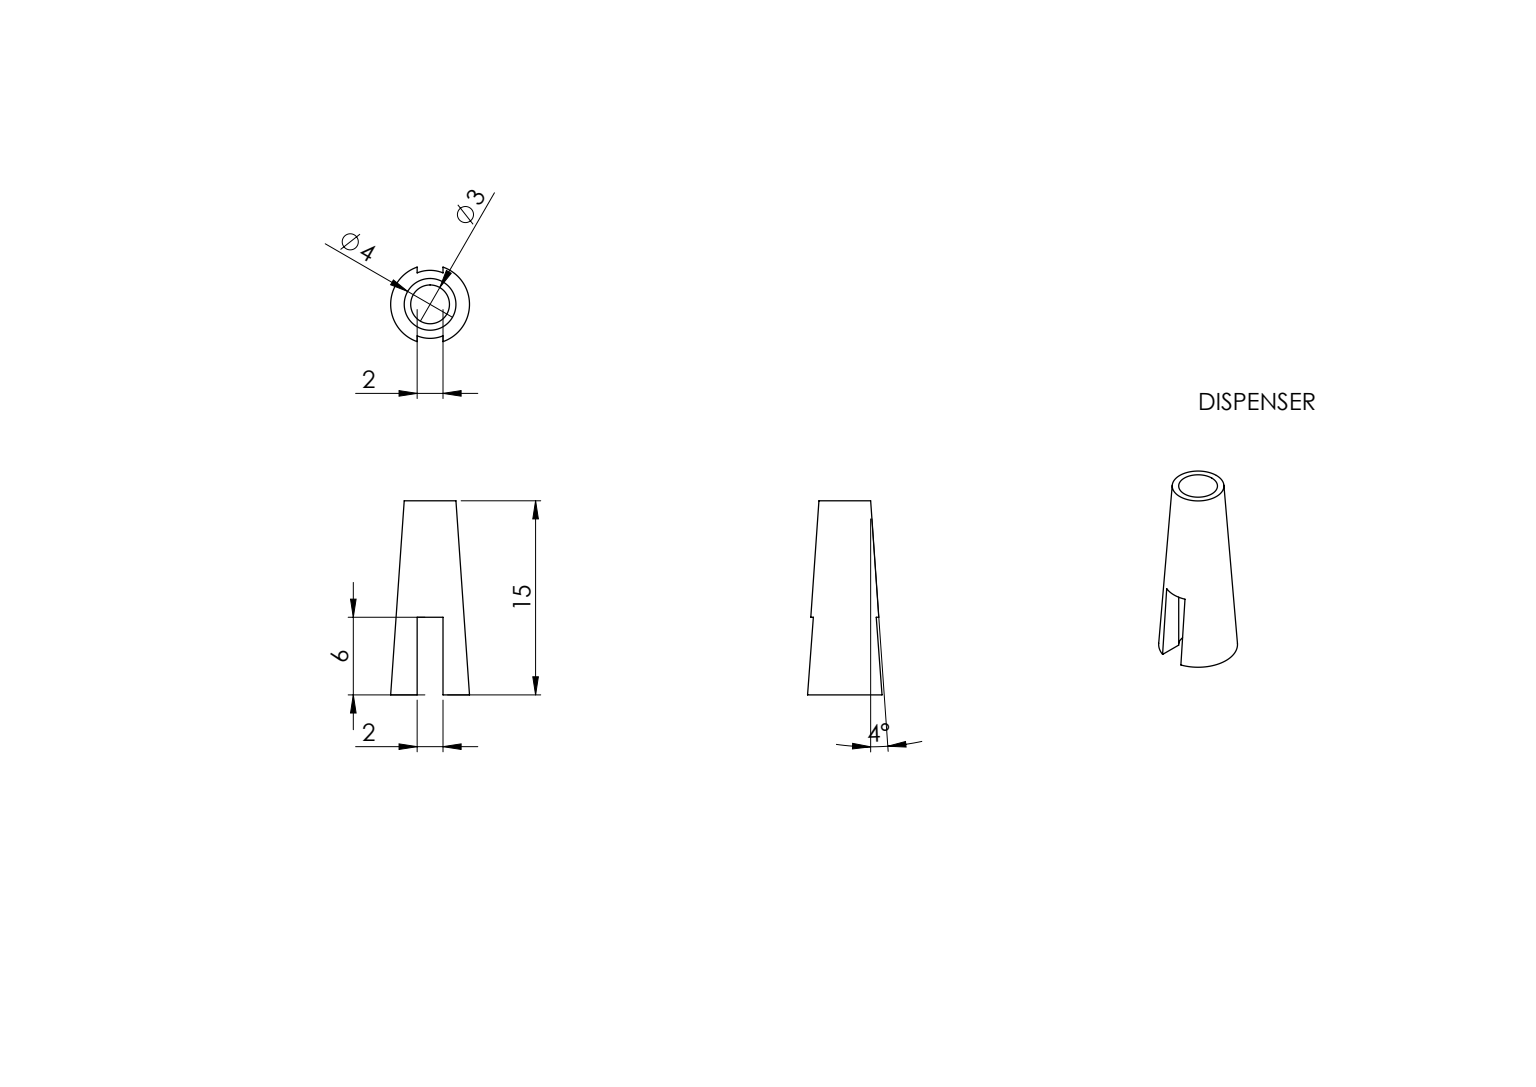
ISO-10303-21;
HEADER;
FILE_DESCRIPTION (('STEP AP214'),
    '1' );
FILE_NAME ('dispenser.step',
    '2026-10-27T10:49:47',
    ( '' ),
    ( '' ),
    'SwSTEP 2.0',
    'SolidWorks 2026',
    '' );
FILE_SCHEMA (( 'AUTOMOTIVE_DESIGN' ));
ENDSEC;

DATA;
#7=CARTESIAN_POINT ( 'NONE',  ( 1.000000000000000000, -30.99987166532831395, 2.582963027349738816 ) ) ;
#10=VECTOR ( 'NONE', #8817, 1000.000000000000000 ) ;
#30=CARTESIAN_POINT ( 'NONE',  ( -1.000000000000000000, -29.00000000000000355, -1.118033988749894680 ) ) ;
#57=DIRECTION ( 'NONE',  ( 0.000000000000000000, 0.000000000000000000, -1.000000000000000000 ) ) ;
#70=CARTESIAN_POINT ( 'NONE',  ( 1.000000000000000000, -29.00000000000000355, -2.431755684948965435 ) ) ;
#75=LINE ( 'NONE', #5700, #8771 ) ;
#80=DIRECTION ( 'NONE',  ( 0.000000000000000000, 0.000000000000000000, -1.000000000000000000 ) ) ;
#99=PRODUCT_DEFINITION_SHAPE ( 'NONE', 'NONE',  #1543 ) ;
#107=CARTESIAN_POINT ( 'NONE',  ( 0.000000000000000000, -29.00000000000000355, -1.499999999999999778 ) ) ;
#115=CARTESIAN_POINT ( 'NONE',  ( 1.836970198721029688E-16, -29.00000000000000355, 1.499999999999999778 ) ) ;
#120=UNCERTAINTY_MEASURE_WITH_UNIT (LENGTH_MEASURE( 1.000000000000000082E-05 ), #327, 'distance_accuracy_value', 'NONE');
#123=CIRCLE ( 'NONE', #1315, 2.629341307491595447 ) ;
#134=FACE_OUTER_BOUND ( 'NONE', #6393, .T. ) ;
#153=DIRECTION ( 'NONE',  ( 1.000000000000000000, 0.000000000000000000, 0.000000000000000000 ) ) ;
#178=DIRECTION ( 'NONE',  ( 0.000000000000000000, -1.000000000000000000, 0.000000000000000000 ) ) ;
#228=FACE_OUTER_BOUND ( 'NONE', #8574, .T. ) ;
#277=ORIENTED_EDGE ( 'NONE', *, *, #3202, .T. ) ;
#282=AXIS2_PLACEMENT_3D ( 'NONE', #7052, #2786, #2167 ) ;
#327=( LENGTH_UNIT ( ) NAMED_UNIT ( * ) SI_UNIT ( .MILLI., .METRE. ) );
#344=AXIS2_PLACEMENT_3D ( 'NONE', #6374, #8568, #2197 ) ;
#388=EDGE_LOOP ( 'NONE', ( #5734, #5832, #6280, #502 ) ) ;
#501=( GEOMETRIC_REPRESENTATION_CONTEXT ( 3 ) GLOBAL_UNCERTAINTY_ASSIGNED_CONTEXT ( ( #1749 ) ) GLOBAL_UNIT_ASSIGNED_CONTEXT ( ( #4938, #8573, #8161 ) ) REPRESENTATION_CONTEXT ( 'NONE', 'WORKASPACE' ) );
#502=ORIENTED_EDGE ( 'NONE', *, *, #1398, .F. ) ;
#521=DIRECTION ( 'NONE',  ( 0.000000000000000000, 0.000000000000000000, -1.000000000000000000 ) ) ;
#574=VECTOR ( 'NONE', #6967, 1000.000000000000000 ) ;
#647=AXIS2_PLACEMENT_3D ( 'NONE', #4691, #1868, #7487 ) ;
#652=EDGE_CURVE ( 'NONE', #8139, #3081, #2009, .T. ) ;
#656=ORIENTED_EDGE ( 'NONE', *, *, #6309, .F. ) ;
#677=ORIENTED_EDGE ( 'NONE', *, *, #5454, .F. ) ;
#678=CARTESIAN_POINT ( 'NONE',  ( -1.000000000000000000, -20.00000000000000000, 1.118033988749894680 ) ) ;
#699=( GEOMETRIC_REPRESENTATION_CONTEXT ( 3 ) GLOBAL_UNCERTAINTY_ASSIGNED_CONTEXT ( ( #120 ) ) GLOBAL_UNIT_ASSIGNED_CONTEXT ( ( #327, #6002, #8152 ) ) REPRESENTATION_CONTEXT ( 'NONE', 'WORKASPACE' ) );
#702=DIRECTION ( 'NONE',  ( 0.000000000000000000, 0.000000000000000000, -1.000000000000000000 ) ) ;
#718=LINE ( 'NONE', #5695, #7261 ) ;
#720=ORIENTED_EDGE ( 'NONE', *, *, #7534, .F. ) ;
#721=DIRECTION ( 'NONE',  ( -0.000000000000000000, -0.000000000000000000, 1.000000000000000000 ) ) ;
#723=DIRECTION ( 'NONE',  ( 1.000000000000000000, 0.000000000000000000, 0.000000000000000000 ) ) ;
#742=CONICAL_SURFACE ( 'NONE', #6530, 2.000000000000000000, 0.06981317007977333455 ) ;
#762=ORIENTED_EDGE ( 'NONE', *, *, #2487, .F. ) ;
#783=EDGE_CURVE ( 'NONE', #3636, #7860, #7922, .T. ) ;
#852=ORIENTED_EDGE ( 'NONE', *, *, #1586, .F. ) ;
#873=CARTESIAN_POINT ( 'NONE',  ( 0.000000000000000000, -29.00000000000000355, 0.000000000000000000 ) ) ;
#883=ORIENTED_EDGE ( 'NONE', *, *, #8729, .F. ) ;
#888=AXIS2_PLACEMENT_3D ( 'NONE', #4026, #9081, #6861 ) ;
#894=CARTESIAN_POINT ( 'NONE',  ( -1.000000000000000000, -30.99987166532831395, 2.582963027349738816 ) ) ;
#950=DIRECTION ( 'NONE',  ( 0.000000000000000000, -1.000000000000000000, 0.000000000000000000 ) ) ;
#997=CARTESIAN_POINT ( 'NONE',  ( -1.000000000000000000, -29.00000000000000355, -3.048902179152658931 ) ) ;
#1022=ORIENTED_EDGE ( 'NONE', *, *, #4471, .T. ) ;
#1029=EDGE_LOOP ( 'NONE', ( #277, #4373, #5520, #6752, #7836, #4879, #5582, #4542 ) ) ;
#1102=DIRECTION ( 'NONE',  ( 0.000000000000000000, -1.000000000000000000, 0.000000000000000000 ) ) ;
#1137=CARTESIAN_POINT ( 'NONE',  ( 0.000000000000000000, -35.00000000000000000, 0.000000000000000000 ) ) ;
#1194=AXIS2_PLACEMENT_3D ( 'NONE', #7137, #7046, #3559 ) ;
#1208=DIRECTION ( 'NONE',  ( 0.000000000000000000, -0.000000000000000000, -1.000000000000000000 ) ) ;
#1241=DIRECTION ( 'NONE',  ( 0.000000000000000000, 0.000000000000000000, -1.000000000000000000 ) ) ;
#1282=EDGE_LOOP ( 'NONE', ( #7453, #8242, #8885, #677 ) ) ;
#1286=VERTEX_POINT ( 'NONE', #30 ) ;
#1307=EDGE_CURVE ( 'NONE', #6715, #7860, #2924, .T. ) ;
#1315=AXIS2_PLACEMENT_3D ( 'NONE', #2177, #2930, #80 ) ;
#1338=AXIS2_PLACEMENT_3D ( 'NONE', #873, #178, #3771 ) ;
#1360=ADVANCED_FACE ( 'NONE', ( #4178, #2747 ), #7806, .F. ) ;
#1387=DIRECTION ( 'NONE',  ( 0.000000000000000000, -0.000000000000000000, -1.000000000000000000 ) ) ;
#1392=CARTESIAN_POINT ( 'NONE',  ( 1.000000000000000000, -29.00000000000000355, 1.118033988749894680 ) ) ;
#1398=EDGE_CURVE ( 'NONE', #6849, #8000, #8214, .T. ) ;
#1409=PLANE ( 'NONE',  #344 ) ;
#1420=DIRECTION ( 'NONE',  ( -0.000000000000000000, -0.000000000000000000, 1.000000000000000000 ) ) ;
#1442=EDGE_CURVE ( 'NONE', #1286, #7860, #7941, .T. ) ;
#1448=CARTESIAN_POINT ( 'NONE',  ( -1.000000000000000000, -35.00000000000000000, -2.880243826144208708 ) ) ;
#1466=CARTESIAN_POINT ( 'NONE',  ( 1.000000000000000000, -35.00000000000000000, -2.880243826144208708 ) ) ;
#1497=DIRECTION ( 'NONE',  ( 0.000000000000000000, 0.000000000000000000, -1.000000000000000000 ) ) ;
#1498=CARTESIAN_POINT ( 'NONE',  ( -1.000000000000000000, -35.00000000000000000, 2.880243826144208708 ) ) ;
#1514=CARTESIAN_POINT ( 'NONE',  ( -1.000000000000000000, -35.00000000000000000, -3.048902179152658931 ) ) ;
#1543=PRODUCT_DEFINITION ( 'UNKNOWN', '', #8579, #8974 ) ;
#1586=EDGE_CURVE ( 'NONE', #7256, #3429, #6249, .T. ) ;
#1590=CARTESIAN_POINT ( 'NONE',  ( 1.000000000000000000, -35.00000000000000000, -1.118033988749894680 ) ) ;
#1591=DIRECTION ( 'NONE',  ( 8.542704229054961664E-18, -0.9975640502598241977, 0.06975647374412545509 ) ) ;
#1637=AXIS2_PLACEMENT_3D ( 'NONE', #1137, #4623, #5581 ) ;
#1638=CARTESIAN_POINT ( 'NONE',  ( 0.000000000000000000, -29.00000000000000355, 0.000000000000000000 ) ) ;
#1644=FACE_OUTER_BOUND ( 'NONE', #1282, .T. ) ;
#1695=DIRECTION ( 'NONE',  ( 1.000000000000000000, 0.000000000000000000, 0.000000000000000000 ) ) ;
#1714=DIRECTION ( 'NONE',  ( 0.000000000000000000, -1.000000000000000000, 0.000000000000000000 ) ) ;
#1749=UNCERTAINTY_MEASURE_WITH_UNIT (LENGTH_MEASURE( 1.000000000000000082E-05 ), #4938, 'distance_accuracy_value', 'NONE');
#1827=SHAPE_REPRESENTATION_RELATIONSHIP ( 'NONE' , 'NONE' ,  #1843, #2088 ) ;
#1834=CYLINDRICAL_SURFACE ( 'NONE', #6978, 1.499999999999999778 ) ;
#1841=CARTESIAN_POINT ( 'NONE',  ( 0.000000000000000000, -20.00000000000000000, 0.000000000000000000 ) ) ;
#1843=SHAPE_REPRESENTATION ( 'dispenser', ( #888 ), #699 ) ;
#1868=DIRECTION ( 'NONE',  ( 0.000000000000000000, -1.000000000000000000, 0.000000000000000000 ) ) ;
#1888=EDGE_CURVE ( 'NONE', #7866, #8580, #8382, .T. ) ;
#1894=CARTESIAN_POINT ( 'NONE',  ( 0.000000000000000000, -20.00000000000000000, 0.000000000000000000 ) ) ;
#1905=MECHANICAL_DESIGN_GEOMETRIC_PRESENTATION_REPRESENTATION('',(#9023),#3833);
#1915=EDGE_CURVE ( 'NONE', #4653, #8235, #4037, .T. ) ;
#1921=DIRECTION ( 'NONE',  ( -0.000000000000000000, -1.000000000000000000, -0.000000000000000000 ) ) ;
#1943=VERTEX_POINT ( 'NONE', #6193 ) ;
#1944=CARTESIAN_POINT ( 'NONE',  ( 0.000000000000000000, -35.00000000000000000, 0.000000000000000000 ) ) ;
#1967=VERTEX_POINT ( 'NONE', #5393 ) ;
#1988=B_SPLINE_CURVE_WITH_KNOTS ( 'NONE', 3,
 ( #6414, #7, #8480, #2810 ),
 .UNSPECIFIED., .F., .F.,
 ( 4, 4 ),
 ( 0.008580651465885628590, 0.01459740681124464291 ),
 .UNSPECIFIED. ) ;
#2009=LINE ( 'NONE', #3362, #3473 ) ;
#2012=SURFACE_STYLE_USAGE ( .BOTH. , #6196 ) ;
#2024=FACE_OUTER_BOUND ( 'NONE', #4217, .T. ) ;
#2088=ADVANCED_BREP_SHAPE_REPRESENTATION ( '', ( #5133, #888 ), #699 ) ;
#2117=VERTEX_POINT ( 'NONE', #2933 ) ;
#2142=VERTEX_POINT ( 'NONE', #1392 ) ;
#2167=DIRECTION ( 'NONE',  ( 0.000000000000000000, 0.000000000000000000, -1.000000000000000000 ) ) ;
#2177=CARTESIAN_POINT ( 'NONE',  ( 0.000000000000000000, -29.00000000000000355, 0.000000000000000000 ) ) ;
#2197=DIRECTION ( 'NONE',  ( 0.000000000000000000, -0.000000000000000000, -1.000000000000000000 ) ) ;
#2198=CARTESIAN_POINT ( 'NONE',  ( 0.000000000000000000, -29.00000000000000355, 0.000000000000000000 ) ) ;
#2211=CARTESIAN_POINT ( 'NONE',  ( 0.000000000000000000, -20.00000000000000000, -1.499999999999999778 ) ) ;
#2221=DIRECTION ( 'NONE',  ( -0.000000000000000000, -0.000000000000000000, 1.000000000000000000 ) ) ;
#2228=CIRCLE ( 'NONE', #3431, 2.629341307491595447 ) ;
#2232=ORIENTED_EDGE ( 'NONE', *, *, #9006, .T. ) ;
#2300=PLANE ( 'NONE',  #4310 ) ;
#2321=CARTESIAN_POINT ( 'NONE',  ( -1.000000000000000000, -35.00000000000000000, 1.118033988749894458 ) ) ;
#2355=CARTESIAN_POINT ( 'NONE',  ( 1.836970198721029688E-16, -20.00000000000000000, 1.499999999999999778 ) ) ;
#2369=EDGE_CURVE ( 'NONE', #3636, #4653, #5653, .T. ) ;
#2370=DIRECTION ( 'NONE',  ( 1.000000000000000000, 0.000000000000000000, 0.000000000000000000 ) ) ;
#2384=CIRCLE ( 'NONE', #1637, 1.499999999999999778 ) ;
#2391=ORIENTED_EDGE ( 'NONE', *, *, #1915, .T. ) ;
#2393=AXIS2_PLACEMENT_3D ( 'NONE', #4264, #5741, #6395 ) ;
#2440=PLANE ( 'NONE',  #3474 ) ;
#2442=ORIENTED_EDGE ( 'NONE', *, *, #1307, .T. ) ;
#2487=EDGE_CURVE ( 'NONE', #6849, #8580, #7097, .T. ) ;
#2550=PLANE ( 'NONE',  #8924 ) ;
#2563=B_SPLINE_CURVE_WITH_KNOTS ( 'NONE', 3,
 ( #6467, #894, #4530, #1498 ),
 .UNSPECIFIED., .F., .F.,
 ( 4, 4 ),
 ( 0.008580651465885628590, 0.01459740681124464291 ),
 .UNSPECIFIED. ) ;
#2579=CONICAL_SURFACE ( 'NONE', #6132, 2.000000000000000000, 0.06981317007977333455 ) ;
#2605=EDGE_CURVE ( 'NONE', #3879, #8235, #2967, .T. ) ;
#2606=ORIENTED_EDGE ( 'NONE', *, *, #5013, .T. ) ;
#2614=PLANE ( 'NONE',  #4076 ) ;
#2629=ORIENTED_EDGE ( 'NONE', *, *, #6612, .T. ) ;
#2645=CARTESIAN_POINT ( 'NONE',  ( 0.000000000000000000, -29.00000000000000355, -2.629341307491595447 ) ) ;
#2670=FILL_AREA_STYLE ('',( #4706 ) ) ;
#2679=CARTESIAN_POINT ( 'NONE',  ( 0.000000000000000000, -20.00000000000000000, 0.000000000000000000 ) ) ;
#2681=FACE_OUTER_BOUND ( 'NONE', #1029, .T. ) ;
#2686=CLOSED_SHELL ( 'NONE', ( #8780, #4900, #2740, #3301, #7354, #1360, #6740, #5728, #3114, #3810, #5162, #9032, #5050 ) ) ;
#2713=VERTEX_POINT ( 'NONE', #2645 ) ;
#2740=ADVANCED_FACE ( 'NONE', ( #8267 ), #2550, .T. ) ;
#2747=FACE_OUTER_BOUND ( 'NONE', #6001, .T. ) ;
#2778=EDGE_CURVE ( 'NONE', #6849, #1943, #8193, .T. ) ;
#2786=DIRECTION ( 'NONE',  ( 0.000000000000000000, -1.000000000000000000, 0.000000000000000000 ) ) ;
#2810=CARTESIAN_POINT ( 'NONE',  ( 1.000000000000000000, -35.00000000000000000, 2.880243826144208708 ) ) ;
#2891=CIRCLE ( 'NONE', #647, 1.499999999999999778 ) ;
#2893=DIRECTION ( 'NONE',  ( -8.881784197001252323E-16, 0.000000000000000000, -1.000000000000000000 ) ) ;
#2896=EDGE_LOOP ( 'NONE', ( #2606, #5966, #5717, #4939 ) ) ;
#2904=APPLICATION_CONTEXT ( 'automotive_design' ) ;
#2924=LINE ( 'NONE', #1514, #574 ) ;
#2925=CARTESIAN_POINT ( 'NONE',  ( 1.000000000000000000, -35.00000000000000000, -3.048902179152658931 ) ) ;
#2930=DIRECTION ( 'NONE',  ( 0.000000000000000000, -1.000000000000000000, 0.000000000000000000 ) ) ;
#2933=CARTESIAN_POINT ( 'NONE',  ( 1.000000000000000000, -35.00000000000000000, 1.118033988749894680 ) ) ;
#2967=LINE ( 'NONE', #2355, #4889 ) ;
#2980=AXIS2_PLACEMENT_3D ( 'NONE', #4346, #5174, #4534 ) ;
#2985=EDGE_CURVE ( 'NONE', #8235, #2142, #6371, .T. ) ;
#2986=DIRECTION ( 'NONE',  ( -0.000000000000000000, -1.000000000000000000, -0.000000000000000000 ) ) ;
#3003=CARTESIAN_POINT ( 'NONE',  ( 1.000000000000000000, -35.00000000000000000, -3.048902179152658931 ) ) ;
#3014=CARTESIAN_POINT ( 'NONE',  ( -1.000000000000000000, -20.00000000000000000, -1.118033988749894680 ) ) ;
#3053=ORIENTED_EDGE ( 'NONE', *, *, #3787, .T. ) ;
#3076=PLANE ( 'NONE',  #8474 ) ;
#3081=VERTEX_POINT ( 'NONE', #107 ) ;
#3096=ORIENTED_EDGE ( 'NONE', *, *, #4416, .F. ) ;
#3114=ADVANCED_FACE ( 'NONE', ( #7272 ), #2300, .T. ) ;
#3128=AXIS2_PLACEMENT_3D ( 'NONE', #2198, #5020, #1497 ) ;
#3148=VECTOR ( 'NONE', #1921, 1000.000000000000000 ) ;
#3202=EDGE_CURVE ( 'NONE', #3429, #7256, #6382, .T. ) ;
#3265=DIRECTION ( 'NONE',  ( -0.000000000000000000, 1.000000000000000000, -0.000000000000000000 ) ) ;
#3267=EDGE_CURVE ( 'NONE', #8580, #2117, #2384, .T. ) ;
#3301=ADVANCED_FACE ( 'NONE', ( #4714 ), #742, .T. ) ;
#3315=CARTESIAN_POINT ( 'NONE',  ( 0.000000000000000000, -20.00000000000000000, 0.000000000000000000 ) ) ;
#3353=CARTESIAN_POINT ( 'NONE',  ( -1.000000000000000000, -29.00000000000000355, -3.048902179152658931 ) ) ;
#3355=PRODUCT_CONTEXT ( 'NONE', #3383, 'mechanical' ) ;
#3362=CARTESIAN_POINT ( 'NONE',  ( 0.000000000000000000, -20.00000000000000000, -1.499999999999999778 ) ) ;
#3383=APPLICATION_CONTEXT ( 'automotive_design' ) ;
#3429=VERTEX_POINT ( 'NONE', #5621 ) ;
#3431=AXIS2_PLACEMENT_3D ( 'NONE', #1638, #6419, #57 ) ;
#3434=ORIENTED_EDGE ( 'NONE', *, *, #3202, .F. ) ;
#3451=EDGE_LOOP ( 'NONE', ( #4192, #3495, #3053, #5205, #8532, #720 ) ) ;
#3473=VECTOR ( 'NONE', #6791, 1000.000000000000000 ) ;
#3474=AXIS2_PLACEMENT_3D ( 'NONE', #3003, #153, #7318 ) ;
#3479=EDGE_CURVE ( 'NONE', #7866, #3081, #7126, .T. ) ;
#3483=CARTESIAN_POINT ( 'NONE',  ( 1.836970198721029688E-16, -20.00000000000000000, 1.499999999999999778 ) ) ;
#3495=ORIENTED_EDGE ( 'NONE', *, *, #7243, .T. ) ;
#3523=PRODUCT ( 'dispenser', 'dispenser', '', ( #3355 ) ) ;
#3550=CYLINDRICAL_SURFACE ( 'NONE', #4735, 1.499999999999999778 ) ;
#3559=DIRECTION ( 'NONE',  ( 0.000000000000000000, 0.000000000000000000, -1.000000000000000000 ) ) ;
#3577=DIRECTION ( 'NONE',  ( 0.000000000000000000, -1.000000000000000000, 0.000000000000000000 ) ) ;
#3596=CARTESIAN_POINT ( 'NONE',  ( -1.000000000000000000, -32.99988997691444581, -2.732192653641477786 ) ) ;
#3636=VERTEX_POINT ( 'NONE', #2321 ) ;
#3660=UNCERTAINTY_MEASURE_WITH_UNIT (LENGTH_MEASURE( 1.000000000000000082E-05 ), #4661, 'distance_accuracy_value', 'NONE');
#3686=LINE ( 'NONE', #6464, #4761 ) ;
#3697=VECTOR ( 'NONE', #2221, 1000.000000000000000 ) ;
#3699=EDGE_LOOP ( 'NONE', ( #3096, #5860, #4421, #656, #6195, #3921, #6067, #6710 ) ) ;
#3771=DIRECTION ( 'NONE',  ( 0.000000000000000000, 0.000000000000000000, -1.000000000000000000 ) ) ;
#3787=EDGE_CURVE ( 'NONE', #8000, #7866, #75, .T. ) ;
#3790=LINE ( 'NONE', #8615, #6417 ) ;
#3810=ADVANCED_FACE ( 'NONE', ( #5611 ), #8458, .F. ) ;
#3814=DIRECTION ( 'NONE',  ( 0.000000000000000000, 0.000000000000000000, -1.000000000000000000 ) ) ;
#3833=( GEOMETRIC_REPRESENTATION_CONTEXT ( 3 ) GLOBAL_UNCERTAINTY_ASSIGNED_CONTEXT ( ( #3660 ) ) GLOBAL_UNIT_ASSIGNED_CONTEXT ( ( #4661, #8978, #5492 ) ) REPRESENTATION_CONTEXT ( 'NONE', 'WORKASPACE' ) );
#3859=CARTESIAN_POINT ( 'NONE',  ( 0.000000000000000000, -35.00000000000000000, 0.000000000000000000 ) ) ;
#3866=CARTESIAN_POINT ( 'NONE',  ( 1.000000000000000000, -35.00000000000000000, -2.880243826144208708 ) ) ;
#3874=AXIS2_PLACEMENT_3D ( 'NONE', #2925, #723, #5792 ) ;
#3879=VERTEX_POINT ( 'NONE', #3483 ) ;
#3882=DIRECTION ( 'NONE',  ( -0.000000000000000000, -1.000000000000000000, -0.000000000000000000 ) ) ;
#3917=EDGE_LOOP ( 'NONE', ( #6738, #2442, #7210, #5313 ) ) ;
#3921=ORIENTED_EDGE ( 'NONE', *, *, #7992, .F. ) ;
#3927=FACE_OUTER_BOUND ( 'NONE', #6004, .T. ) ;
#3928=CARTESIAN_POINT ( 'NONE',  ( -1.000000000000000000, -29.00000000000000355, -2.431755684948965435 ) ) ;
#3950=EDGE_CURVE ( 'NONE', #3429, #2713, #3686, .T. ) ;
#3977=DIRECTION ( 'NONE',  ( 0.000000000000000000, 0.000000000000000000, -1.000000000000000000 ) ) ;
#4000=VECTOR ( 'NONE', #5364, 1000.000000000000000 ) ;
#4009=VERTEX_POINT ( 'NONE', #7875 ) ;
#4023=EDGE_CURVE ( 'NONE', #6825, #6014, #2228, .T. ) ;
#4026=CARTESIAN_POINT ( 'NONE',  ( 0.000000000000000000, 0.000000000000000000, 0.000000000000000000 ) ) ;
#4037=CIRCLE ( 'NONE', #4321, 1.499999999999999778 ) ;
#4076=AXIS2_PLACEMENT_3D ( 'NONE', #3353, #5431, #1208 ) ;
#4178=FACE_BOUND ( 'NONE', #5344, .T. ) ;
#4180=AXIS2_PLACEMENT_3D ( 'NONE', #1944, #1102, #1241 ) ;
#4185=CARTESIAN_POINT ( 'NONE',  ( 3.091560946453699876E-16, -20.00000000000000000, 2.000000000000000000 ) ) ;
#4192=ORIENTED_EDGE ( 'NONE', *, *, #6309, .T. ) ;
#4213=ORIENTED_EDGE ( 'NONE', *, *, #8224, .T. ) ;
#4217=EDGE_LOOP ( 'NONE', ( #8444, #2232, #8112, #2391, #6761, #5078 ) ) ;
#4264=CARTESIAN_POINT ( 'NONE',  ( 0.000000000000000000, -20.00000000000000000, 0.000000000000000000 ) ) ;
#4270=CARTESIAN_POINT ( 'NONE',  ( 1.000000000000000000, -29.00000000000000355, -3.048902179152658931 ) ) ;
#4292=CARTESIAN_POINT ( 'NONE',  ( -1.000000000000000000, -30.99986970103996953, -2.582962878832828046 ) ) ;
#4310=AXIS2_PLACEMENT_3D ( 'NONE', #8017, #1695, #5778 ) ;
#4312=CARTESIAN_POINT ( 'NONE',  ( 1.000000000000000000, -30.99986970103996953, -2.582962878832828046 ) ) ;
#4321=AXIS2_PLACEMENT_3D ( 'NONE', #4747, #3265, #521 ) ;
#4346=CARTESIAN_POINT ( 'NONE',  ( 0.000000000000000000, -20.00000000000000000, 0.000000000000000000 ) ) ;
#4356=LINE ( 'NONE', #997, #8596 ) ;
#4373=ORIENTED_EDGE ( 'NONE', *, *, #4416, .T. ) ;
#4416=EDGE_CURVE ( 'NONE', #7256, #6014, #3790, .T. ) ;
#4421=ORIENTED_EDGE ( 'NONE', *, *, #3950, .T. ) ;
#4471=EDGE_CURVE ( 'NONE', #4009, #1967, #2563, .T. ) ;
#4508=AXIS2_PLACEMENT_3D ( 'NONE', #3859, #1714, #5148 ) ;
#4530=CARTESIAN_POINT ( 'NONE',  ( -1.000000000000000000, -32.99989163573538775, 2.732192776429915426 ) ) ;
#4533=EDGE_LOOP ( 'NONE', ( #762, #5883, #6020, #7756 ) ) ;
#4534=DIRECTION ( 'NONE',  ( 0.000000000000000000, 0.000000000000000000, -1.000000000000000000 ) ) ;
#4542=ORIENTED_EDGE ( 'NONE', *, *, #3950, .F. ) ;
#4623=DIRECTION ( 'NONE',  ( 0.000000000000000000, -1.000000000000000000, 0.000000000000000000 ) ) ;
#4653=VERTEX_POINT ( 'NONE', #6855 ) ;
#4661=( LENGTH_UNIT ( ) NAMED_UNIT ( * ) SI_UNIT ( .MILLI., .METRE. ) );
#4663=VERTEX_POINT ( 'NONE', #3928 ) ;
#4670=DIRECTION ( 'NONE',  ( 0.000000000000000000, -1.000000000000000000, 0.000000000000000000 ) ) ;
#4691=CARTESIAN_POINT ( 'NONE',  ( 0.000000000000000000, -20.00000000000000000, 0.000000000000000000 ) ) ;
#4706=FILL_AREA_STYLE_COLOUR ( '', #7840 ) ;
#4714=FACE_OUTER_BOUND ( 'NONE', #3699, .T. ) ;
#4735=AXIS2_PLACEMENT_3D ( 'NONE', #2679, #2986, #702 ) ;
#4747=CARTESIAN_POINT ( 'NONE',  ( 0.000000000000000000, -29.00000000000000355, 0.000000000000000000 ) ) ;
#4751=CIRCLE ( 'NONE', #3128, 1.499999999999999778 ) ;
#4761=VECTOR ( 'NONE', #5865, 1000.000000000000227 ) ;
#4780=CARTESIAN_POINT ( 'NONE',  ( 1.000000000000000000, -29.00000000000000355, -1.118033988749894680 ) ) ;
#4877=AXIS2_PLACEMENT_3D ( 'NONE', #7765, #3577, #1387 ) ;
#4879=ORIENTED_EDGE ( 'NONE', *, *, #1398, .T. ) ;
#4889=VECTOR ( 'NONE', #5790, 1000.000000000000000 ) ;
#4900=ADVANCED_FACE ( 'NONE', ( #2681 ), #2579, .T. ) ;
#4905=AXIS2_PLACEMENT_3D ( 'NONE', #3315, #6000, #7353 ) ;
#4911=VECTOR ( 'NONE', #7010, 1000.000000000000000 ) ;
#4938=( LENGTH_UNIT ( ) NAMED_UNIT ( * ) SI_UNIT ( .MILLI., .METRE. ) );
#4939=ORIENTED_EDGE ( 'NONE', *, *, #1307, .F. ) ;
#4943=AXIS2_PLACEMENT_3D ( 'NONE', #7323, #950, #7935 ) ;
#5013=EDGE_CURVE ( 'NONE', #6715, #4663, #8093, .T. ) ;
#5020=DIRECTION ( 'NONE',  ( -0.000000000000000000, 1.000000000000000000, -0.000000000000000000 ) ) ;
#5036=ORIENTED_EDGE ( 'NONE', *, *, #2605, .F. ) ;
#5037=AXIS2_PLACEMENT_3D ( 'NONE', #8514, #7950, #2893 ) ;
#5050=ADVANCED_FACE ( 'NONE', ( #2024 ), #1409, .T. ) ;
#5078=ORIENTED_EDGE ( 'NONE', *, *, #7298, .T. ) ;
#5133=MANIFOLD_SOLID_BREP ( 'Cut-Extrude-Thin1', #2686 ) ;
#5148=DIRECTION ( 'NONE',  ( 0.000000000000000000, 0.000000000000000000, -1.000000000000000000 ) ) ;
#5162=ADVANCED_FACE ( 'NONE', ( #1644 ), #2440, .F. ) ;
#5174=DIRECTION ( 'NONE',  ( 0.000000000000000000, -1.000000000000000000, 0.000000000000000000 ) ) ;
#5205=ORIENTED_EDGE ( 'NONE', *, *, #3479, .T. ) ;
#5250=CARTESIAN_POINT ( 'NONE',  ( 1.000000000000000000, -29.00000000000000355, 2.431755684948965435 ) ) ;
#5263=CARTESIAN_POINT ( 'NONE',  ( 0.000000000000000000, -20.00000000000000000, 0.000000000000000000 ) ) ;
#5267=ORIENTED_EDGE ( 'NONE', *, *, #2369, .F. ) ;
#5297=ORIENTED_EDGE ( 'NONE', *, *, #1915, .F. ) ;
#5313=ORIENTED_EDGE ( 'NONE', *, *, #7954, .T. ) ;
#5344=EDGE_LOOP ( 'NONE', ( #8996, #7140 ) ) ;
#5364=DIRECTION ( 'NONE',  ( 0.000000000000000000, 1.000000000000000000, 0.000000000000000000 ) ) ;
#5375=ORIENTED_EDGE ( 'NONE', *, *, #1442, .F. ) ;
#5393=CARTESIAN_POINT ( 'NONE',  ( -1.000000000000000000, -35.00000000000000000, 2.880243826144208708 ) ) ;
#5431=DIRECTION ( 'NONE',  ( 0.000000000000000000, -1.000000000000000000, 0.000000000000000000 ) ) ;
#5454=EDGE_CURVE ( 'NONE', #6825, #1943, #1988, .T. ) ;
#5456=CARTESIAN_POINT ( 'NONE',  ( 0.000000000000000000, -20.00000000000000000, 0.000000000000000000 ) ) ;
#5466=CARTESIAN_POINT ( 'NONE',  ( 0.000000000000000000, -35.00000000000000000, 0.000000000000000000 ) ) ;
#5492=( NAMED_UNIT ( * ) SI_UNIT ( $, .STERADIAN. ) SOLID_ANGLE_UNIT ( ) );
#5520=ORIENTED_EDGE ( 'NONE', *, *, #4023, .F. ) ;
#5552=DIRECTION ( 'NONE',  ( 0.000000000000000000, 0.000000000000000000, -1.000000000000000000 ) ) ;
#5558=ORIENTED_EDGE ( 'NONE', *, *, #1888, .T. ) ;
#5581=DIRECTION ( 'NONE',  ( 0.000000000000000000, 0.000000000000000000, -1.000000000000000000 ) ) ;
#5582=ORIENTED_EDGE ( 'NONE', *, *, #7243, .F. ) ;
#5603=ORIENTED_EDGE ( 'NONE', *, *, #3267, .T. ) ;
#5611=FACE_OUTER_BOUND ( 'NONE', #388, .T. ) ;
#5621=CARTESIAN_POINT ( 'NONE',  ( 0.000000000000000000, -20.00000000000000000, -2.000000000000000000 ) ) ;
#5641=CIRCLE ( 'NONE', #1338, 2.629341307491595447 ) ;
#5651=LINE ( 'NONE', #6266, #6509 ) ;
#5653=LINE ( 'NONE', #678, #4911 ) ;
#5680=CARTESIAN_POINT ( 'NONE',  ( -1.000000000000000000, -29.00000000000000355, -2.431755684948965435 ) ) ;
#5692=ORIENTED_EDGE ( 'NONE', *, *, #7954, .F. ) ;
#5695=CARTESIAN_POINT ( 'NONE',  ( -1.000000000000000000, -35.00000000000000000, -3.048902179152658931 ) ) ;
#5700=CARTESIAN_POINT ( 'NONE',  ( 1.000000000000000000, -29.00000000000000355, -3.048902179152658931 ) ) ;
#5709=EDGE_CURVE ( 'NONE', #3879, #8139, #2891, .T. ) ;
#5717=ORIENTED_EDGE ( 'NONE', *, *, #1442, .T. ) ;
#5728=ADVANCED_FACE ( 'NONE', ( #9011 ), #2614, .T. ) ;
#5734=ORIENTED_EDGE ( 'NONE', *, *, #2487, .T. ) ;
#5739=ORIENTED_EDGE ( 'NONE', *, *, #2369, .T. ) ;
#5741=DIRECTION ( 'NONE',  ( 0.000000000000000000, -1.000000000000000000, 0.000000000000000000 ) ) ;
#5778=DIRECTION ( 'NONE',  ( 0.000000000000000000, 0.000000000000000000, -1.000000000000000000 ) ) ;
#5790=DIRECTION ( 'NONE',  ( -0.000000000000000000, -1.000000000000000000, -0.000000000000000000 ) ) ;
#5792=DIRECTION ( 'NONE',  ( 0.000000000000000000, 0.000000000000000000, -1.000000000000000000 ) ) ;
#5832=ORIENTED_EDGE ( 'NONE', *, *, #1888, .F. ) ;
#5860=ORIENTED_EDGE ( 'NONE', *, *, #1586, .T. ) ;
#5865=DIRECTION ( 'NONE',  ( 0.000000000000000000, -0.9975640502598241977, -0.06975647374412545509 ) ) ;
#5883=ORIENTED_EDGE ( 'NONE', *, *, #2778, .T. ) ;
#5897=CARTESIAN_POINT ( 'NONE',  ( -1.000000000000000000, -35.00000000000000000, -3.048902179152658931 ) ) ;
#5939=LINE ( 'NONE', #8779, #8752 ) ;
#5966=ORIENTED_EDGE ( 'NONE', *, *, #7534, .T. ) ;
#5984=STYLED_ITEM('',(#9218),#5133);
#6000=DIRECTION ( 'NONE',  ( 0.000000000000000000, -1.000000000000000000, 0.000000000000000000 ) ) ;
#6001=EDGE_LOOP ( 'NONE', ( #3434, #852 ) ) ;
#6002=( NAMED_UNIT ( * ) PLANE_ANGLE_UNIT ( ) SI_UNIT ( $, .RADIAN. ) );
#6004=EDGE_LOOP ( 'NONE', ( #6955, #7441, #5297, #5267, #7595, #5375, #883, #6048 ) ) ;
#6014=VERTEX_POINT ( 'NONE', #6354 ) ;
#6020=ORIENTED_EDGE ( 'NONE', *, *, #7988, .F. ) ;
#6048=ORIENTED_EDGE ( 'NONE', *, *, #652, .F. ) ;
#6067=ORIENTED_EDGE ( 'NONE', *, *, #4471, .F. ) ;
#6132=AXIS2_PLACEMENT_3D ( 'NONE', #1894, #9085, #5552 ) ;
#6185=SHAPE_DEFINITION_REPRESENTATION ( #99, #1843 ) ;
#6193=CARTESIAN_POINT ( 'NONE',  ( 1.000000000000000000, -35.00000000000000000, 2.880243826144208708 ) ) ;
#6195=ORIENTED_EDGE ( 'NONE', *, *, #5013, .F. ) ;
#6196=SURFACE_SIDE_STYLE ('',( #8291 ) ) ;
#6249=CIRCLE ( 'NONE', #4905, 2.000000000000000000 ) ;
#6266=CARTESIAN_POINT ( 'NONE',  ( 1.000000000000000000, -35.00000000000000000, -3.048902179152658931 ) ) ;
#6280=ORIENTED_EDGE ( 'NONE', *, *, #3787, .F. ) ;
#6309=EDGE_CURVE ( 'NONE', #4663, #2713, #7492, .T. ) ;
#6354=CARTESIAN_POINT ( 'NONE',  ( 3.220014416085498963E-16, -29.00000000000000355, 2.629341307491595447 ) ) ;
#6371=CIRCLE ( 'NONE', #1194, 1.499999999999999778 ) ;
#6374=CARTESIAN_POINT ( 'NONE',  ( -1.000000000000000000, -29.00000000000000355, -3.048902179152658931 ) ) ;
#6382=CIRCLE ( 'NONE', #2980, 2.000000000000000000 ) ;
#6393=EDGE_LOOP ( 'NONE', ( #5036, #7164, #8692, #7547, #5558, #5603, #2629, #6811 ) ) ;
#6395=DIRECTION ( 'NONE',  ( 0.000000000000000000, -0.000000000000000000, -1.000000000000000000 ) ) ;
#6414=CARTESIAN_POINT ( 'NONE',  ( 1.000000000000000000, -29.00000000000000355, 2.431755684948965435 ) ) ;
#6417=VECTOR ( 'NONE', #1591, 1000.000000000000227 ) ;
#6419=DIRECTION ( 'NONE',  ( 0.000000000000000000, -1.000000000000000000, 0.000000000000000000 ) ) ;
#6464=CARTESIAN_POINT ( 'NONE',  ( 0.000000000000000000, -20.00000000000000000, -2.000000000000000000 ) ) ;
#6467=CARTESIAN_POINT ( 'NONE',  ( -1.000000000000000000, -29.00000000000000355, 2.431755684948965435 ) ) ;
#6509=VECTOR ( 'NONE', #8540, 1000.000000000000000 ) ;
#6530=AXIS2_PLACEMENT_3D ( 'NONE', #1841, #4670, #3977 ) ;
#6612=EDGE_CURVE ( 'NONE', #2117, #2142, #7466, .T. ) ;
#6710=ORIENTED_EDGE ( 'NONE', *, *, #9006, .F. ) ;
#6715=VERTEX_POINT ( 'NONE', #9127 ) ;
#6738=ORIENTED_EDGE ( 'NONE', *, *, #7992, .T. ) ;
#6740=ADVANCED_FACE ( 'NONE', ( #134 ), #3550, .F. ) ;
#6752=ORIENTED_EDGE ( 'NONE', *, *, #5454, .T. ) ;
#6761=ORIENTED_EDGE ( 'NONE', *, *, #2985, .T. ) ;
#6769=DIRECTION ( 'NONE',  ( 0.000000000000000000, -1.000000000000000000, 0.000000000000000000 ) ) ;
#6791=DIRECTION ( 'NONE',  ( -0.000000000000000000, -1.000000000000000000, -0.000000000000000000 ) ) ;
#6792=CARTESIAN_POINT ( 'NONE',  ( 1.000000000000000000, -20.00000000000000000, -1.118033988749894680 ) ) ;
#6811=ORIENTED_EDGE ( 'NONE', *, *, #2985, .F. ) ;
#6825=VERTEX_POINT ( 'NONE', #5250 ) ;
#6849=VERTEX_POINT ( 'NONE', #3866 ) ;
#6855=CARTESIAN_POINT ( 'NONE',  ( -1.000000000000000000, -29.00000000000000355, 1.118033988749894680 ) ) ;
#6861=DIRECTION ( 'NONE',  ( 1.000000000000000000, 0.000000000000000000, 0.000000000000000000 ) ) ;
#6891=MECHANICAL_DESIGN_GEOMETRIC_PRESENTATION_REPRESENTATION('',(#5984),#501);
#6955=ORIENTED_EDGE ( 'NONE', *, *, #5709, .F. ) ;
#6967=DIRECTION ( 'NONE',  ( -0.000000000000000000, -0.000000000000000000, 1.000000000000000000 ) ) ;
#6978=AXIS2_PLACEMENT_3D ( 'NONE', #5263, #3882, #7505 ) ;
#6981=VECTOR ( 'NONE', #721, 1000.000000000000000 ) ;
#7010=DIRECTION ( 'NONE',  ( 0.000000000000000000, 1.000000000000000000, 0.000000000000000000 ) ) ;
#7046=DIRECTION ( 'NONE',  ( -0.000000000000000000, 1.000000000000000000, -0.000000000000000000 ) ) ;
#7052=CARTESIAN_POINT ( 'NONE',  ( 0.000000000000000000, -35.00000000000000000, 0.000000000000000000 ) ) ;
#7097=LINE ( 'NONE', #9143, #6981 ) ;
#7106=FACE_OUTER_BOUND ( 'NONE', #4533, .T. ) ;
#7126=CIRCLE ( 'NONE', #5037, 1.499999999999999778 ) ;
#7137=CARTESIAN_POINT ( 'NONE',  ( 0.000000000000000000, -29.00000000000000355, 0.000000000000000000 ) ) ;
#7140=ORIENTED_EDGE ( 'NONE', *, *, #5709, .T. ) ;
#7164=ORIENTED_EDGE ( 'NONE', *, *, #9163, .F. ) ;
#7210=ORIENTED_EDGE ( 'NONE', *, *, #783, .F. ) ;
#7243=EDGE_CURVE ( 'NONE', #2713, #8000, #123, .T. ) ;
#7256=VERTEX_POINT ( 'NONE', #4185 ) ;
#7261=VECTOR ( 'NONE', #1420, 1000.000000000000000 ) ;
#7272=FACE_OUTER_BOUND ( 'NONE', #2896, .T. ) ;
#7276=CIRCLE ( 'NONE', #8907, 1.499999999999999778 ) ;
#7280=DIRECTION ( 'NONE',  ( -0.000000000000000000, -0.000000000000000000, 1.000000000000000000 ) ) ;
#7292=DIRECTION ( 'NONE',  ( -0.000000000000000000, -0.000000000000000000, 1.000000000000000000 ) ) ;
#7298=EDGE_CURVE ( 'NONE', #2142, #6825, #9150, .T. ) ;
#7318=DIRECTION ( 'NONE',  ( 0.000000000000000000, 0.000000000000000000, -1.000000000000000000 ) ) ;
#7323=CARTESIAN_POINT ( 'NONE',  ( 0.000000000000000000, -29.00000000000000355, 0.000000000000000000 ) ) ;
#7353=DIRECTION ( 'NONE',  ( 0.000000000000000000, 0.000000000000000000, -1.000000000000000000 ) ) ;
#7354=ADVANCED_FACE ( 'NONE', ( #7106 ), #8464, .T. ) ;
#7441=ORIENTED_EDGE ( 'NONE', *, *, #2605, .T. ) ;
#7453=ORIENTED_EDGE ( 'NONE', *, *, #7298, .F. ) ;
#7466=LINE ( 'NONE', #8260, #4000 ) ;
#7472=DIRECTION ( 'NONE',  ( 0.000000000000000000, -0.000000000000000000, -1.000000000000000000 ) ) ;
#7487=DIRECTION ( 'NONE',  ( 0.000000000000000000, 0.000000000000000000, -1.000000000000000000 ) ) ;
#7492=CIRCLE ( 'NONE', #4943, 2.629341307491595447 ) ;
#7505=DIRECTION ( 'NONE',  ( 0.000000000000000000, 0.000000000000000000, -1.000000000000000000 ) ) ;
#7534=EDGE_CURVE ( 'NONE', #4663, #1286, #5939, .T. ) ;
#7547=ORIENTED_EDGE ( 'NONE', *, *, #3479, .F. ) ;
#7595=ORIENTED_EDGE ( 'NONE', *, *, #783, .T. ) ;
#7639=PRESENTATION_STYLE_ASSIGNMENT (( #2012 ) ) ;
#7756=ORIENTED_EDGE ( 'NONE', *, *, #3267, .F. ) ;
#7765=CARTESIAN_POINT ( 'NONE',  ( 0.000000000000000000, -35.00000000000000000, 0.000000000000000000 ) ) ;
#7806=PLANE ( 'NONE',  #2393 ) ;
#7836=ORIENTED_EDGE ( 'NONE', *, *, #2778, .F. ) ;
#7840=COLOUR_RGB ( '',0.8941176470588234615, 0.8941176470588234615, 0.8941176470588234615 ) ;
#7860=VERTEX_POINT ( 'NONE', #8321 ) ;
#7866=VERTEX_POINT ( 'NONE', #4780 ) ;
#7875=CARTESIAN_POINT ( 'NONE',  ( -1.000000000000000000, -29.00000000000000355, 2.431755684948965435 ) ) ;
#7922=CIRCLE ( 'NONE', #4508, 1.499999999999999778 ) ;
#7935=DIRECTION ( 'NONE',  ( 0.000000000000000000, 0.000000000000000000, -1.000000000000000000 ) ) ;
#7941=LINE ( 'NONE', #3014, #10 ) ;
#7950=DIRECTION ( 'NONE',  ( -0.000000000000000000, 1.000000000000000000, -0.000000000000000000 ) ) ;
#7954=EDGE_CURVE ( 'NONE', #3636, #1967, #718, .T. ) ;
#7988=EDGE_CURVE ( 'NONE', #2117, #1943, #5651, .T. ) ;
#7992=EDGE_CURVE ( 'NONE', #1967, #6715, #8317, .T. ) ;
#8000=VERTEX_POINT ( 'NONE', #70 ) ;
#8017=CARTESIAN_POINT ( 'NONE',  ( -1.000000000000000000, -35.00000000000000000, -3.048902179152658931 ) ) ;
#8093=B_SPLINE_CURVE_WITH_KNOTS ( 'NONE', 3,
 ( #1448, #3596, #4292, #5680 ),
 .UNSPECIFIED., .F., .F.,
 ( 4, 4 ),
 ( 0.008577873411363935718, 0.01459462325714742936 ),
 .UNSPECIFIED. ) ;
#8112=ORIENTED_EDGE ( 'NONE', *, *, #8224, .F. ) ;
#8139=VERTEX_POINT ( 'NONE', #2211 ) ;
#8152=( NAMED_UNIT ( * ) SI_UNIT ( $, .STERADIAN. ) SOLID_ANGLE_UNIT ( ) );
#8161=( NAMED_UNIT ( * ) SI_UNIT ( $, .STERADIAN. ) SOLID_ANGLE_UNIT ( ) );
#8193=CIRCLE ( 'NONE', #4180, 3.048902179152658931 ) ;
#8214=B_SPLINE_CURVE_WITH_KNOTS ( 'NONE', 3,
 ( #1466, #8586, #4312, #8413 ),
 .UNSPECIFIED., .F., .F.,
 ( 4, 4 ),
 ( 0.008577873411363935718, 0.01459462325714742936 ),
 .UNSPECIFIED. ) ;
#8224=EDGE_CURVE ( 'NONE', #4653, #4009, #4356, .T. ) ;
#8235=VERTEX_POINT ( 'NONE', #115 ) ;
#8242=ORIENTED_EDGE ( 'NONE', *, *, #6612, .F. ) ;
#8260=CARTESIAN_POINT ( 'NONE',  ( 1.000000000000000000, -20.00000000000000000, 1.118033988749894680 ) ) ;
#8267=FACE_OUTER_BOUND ( 'NONE', #3917, .T. ) ;
#8291=SURFACE_STYLE_FILL_AREA ( #2670 ) ;
#8301=DIRECTION ( 'NONE',  ( 0.000000000000000000, -1.000000000000000000, 0.000000000000000000 ) ) ;
#8317=CIRCLE ( 'NONE', #282, 3.048902179152658931 ) ;
#8321=CARTESIAN_POINT ( 'NONE',  ( -1.000000000000000000, -35.00000000000000000, -1.118033988749894680 ) ) ;
#8382=LINE ( 'NONE', #6792, #3148 ) ;
#8413=CARTESIAN_POINT ( 'NONE',  ( 1.000000000000000000, -29.00000000000000355, -2.431755684948965435 ) ) ;
#8444=ORIENTED_EDGE ( 'NONE', *, *, #4023, .T. ) ;
#8458=PLANE ( 'NONE',  #3874 ) ;
#8464=PLANE ( 'NONE',  #4877 ) ;
#8474=AXIS2_PLACEMENT_3D ( 'NONE', #5897, #2370, #3814 ) ;
#8480=CARTESIAN_POINT ( 'NONE',  ( 1.000000000000000000, -32.99989163573538775, 2.732192776429915426 ) ) ;
#8514=CARTESIAN_POINT ( 'NONE',  ( 0.000000000000000000, -29.00000000000000355, 0.000000000000000000 ) ) ;
#8532=ORIENTED_EDGE ( 'NONE', *, *, #8729, .T. ) ;
#8540=DIRECTION ( 'NONE',  ( -0.000000000000000000, -0.000000000000000000, 1.000000000000000000 ) ) ;
#8568=DIRECTION ( 'NONE',  ( 0.000000000000000000, -1.000000000000000000, 0.000000000000000000 ) ) ;
#8573=( NAMED_UNIT ( * ) PLANE_ANGLE_UNIT ( ) SI_UNIT ( $, .RADIAN. ) );
#8574=EDGE_LOOP ( 'NONE', ( #1022, #5692, #5739, #4213 ) ) ;
#8579=PRODUCT_DEFINITION_FORMATION_WITH_SPECIFIED_SOURCE ( 'ANY', '', #3523, .NOT_KNOWN. ) ;
#8580=VERTEX_POINT ( 'NONE', #1590 ) ;
#8586=CARTESIAN_POINT ( 'NONE',  ( 1.000000000000000000, -32.99988997691444581, -2.732192653641477786 ) ) ;
#8596=VECTOR ( 'NONE', #7280, 1000.000000000000000 ) ;
#8615=CARTESIAN_POINT ( 'NONE',  ( 2.449293598294706414E-16, -20.00000000000000000, 2.000000000000000000 ) ) ;
#8692=ORIENTED_EDGE ( 'NONE', *, *, #652, .T. ) ;
#8729=EDGE_CURVE ( 'NONE', #3081, #1286, #4751, .T. ) ;
#8752=VECTOR ( 'NONE', #7292, 1000.000000000000000 ) ;
#8771=VECTOR ( 'NONE', #9145, 1000.000000000000000 ) ;
#8779=CARTESIAN_POINT ( 'NONE',  ( -1.000000000000000000, -29.00000000000000355, -3.048902179152658931 ) ) ;
#8780=ADVANCED_FACE ( 'NONE', ( #3927 ), #1834, .F. ) ;
#8817=DIRECTION ( 'NONE',  ( -0.000000000000000000, -1.000000000000000000, -0.000000000000000000 ) ) ;
#8885=ORIENTED_EDGE ( 'NONE', *, *, #7988, .T. ) ;
#8907=AXIS2_PLACEMENT_3D ( 'NONE', #5456, #8301, #9124 ) ;
#8924=AXIS2_PLACEMENT_3D ( 'NONE', #5466, #6769, #7472 ) ;
#8974=PRODUCT_DEFINITION_CONTEXT ( 'detailed design', #2904, 'design' ) ;
#8978=( NAMED_UNIT ( * ) PLANE_ANGLE_UNIT ( ) SI_UNIT ( $, .RADIAN. ) );
#8996=ORIENTED_EDGE ( 'NONE', *, *, #9163, .T. ) ;
#9006=EDGE_CURVE ( 'NONE', #6014, #4009, #5641, .T. ) ;
#9011=FACE_OUTER_BOUND ( 'NONE', #3451, .T. ) ;
#9023=STYLED_ITEM ( 'NONE', ( #7639 ), #2088 ) ;
#9032=ADVANCED_FACE ( 'NONE', ( #228 ), #3076, .T. ) ;
#9081=DIRECTION ( 'NONE',  ( 0.000000000000000000, 0.000000000000000000, 1.000000000000000000 ) ) ;
#9085=DIRECTION ( 'NONE',  ( 0.000000000000000000, -1.000000000000000000, 0.000000000000000000 ) ) ;
#9124=DIRECTION ( 'NONE',  ( 0.000000000000000000, 0.000000000000000000, -1.000000000000000000 ) ) ;
#9127=CARTESIAN_POINT ( 'NONE',  ( -1.000000000000000000, -35.00000000000000000, -2.880243826144208708 ) ) ;
#9143=CARTESIAN_POINT ( 'NONE',  ( 1.000000000000000000, -35.00000000000000000, -3.048902179152658931 ) ) ;
#9145=DIRECTION ( 'NONE',  ( -0.000000000000000000, -0.000000000000000000, 1.000000000000000000 ) ) ;
#9150=LINE ( 'NONE', #4270, #3697 ) ;
#9163=EDGE_CURVE ( 'NONE', #8139, #3879, #7276, .T. ) ;
#9212=COLOUR_RGB('Sky Blue',0.24,0.69,0.87);
#9213=FILL_AREA_STYLE_COLOUR('',#9212);
#9214=FILL_AREA_STYLE('',(#9213));
#9215=SURFACE_STYLE_FILL_AREA(#9214);
#9216=SURFACE_SIDE_STYLE('',(#9215));
#9217=SURFACE_STYLE_USAGE(.BOTH.,#9216);
#9218=PRESENTATION_STYLE_ASSIGNMENT((#9217));
ENDSEC;
END-ISO-10303-21;
